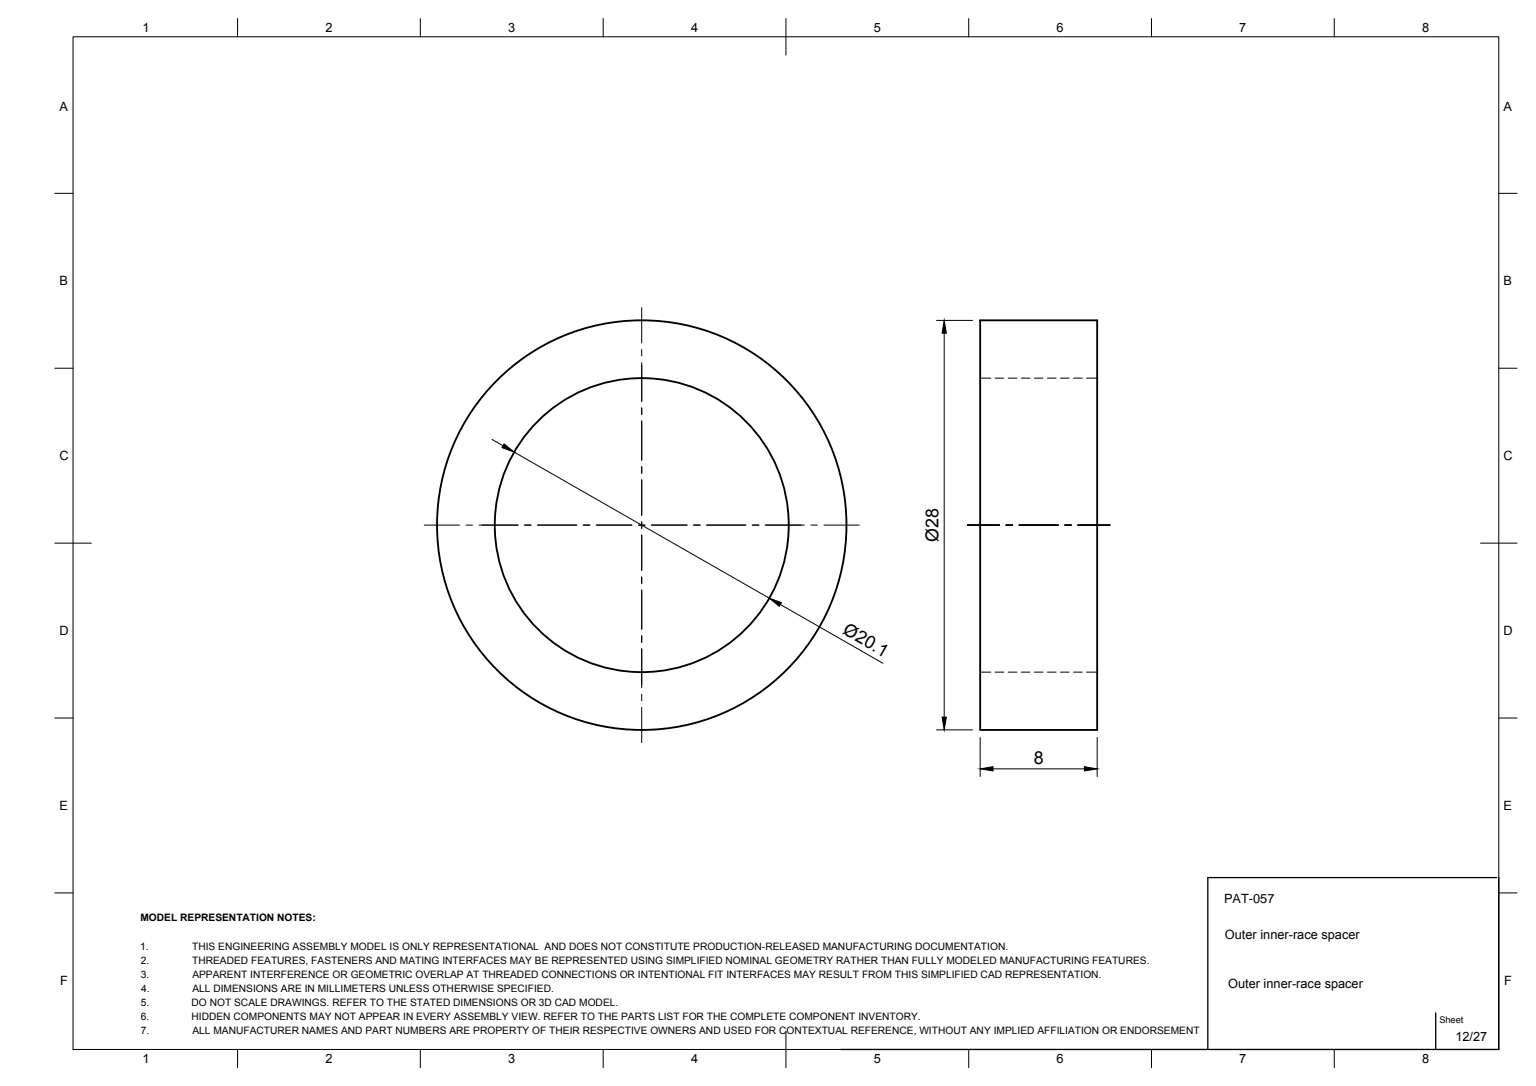
ISO-10303-21;
HEADER;
/* Generated by software containing ST-Developer
 * from STEP Tools, Inc. (www.steptools.com) 
 */

FILE_DESCRIPTION(
/* description */ ('Bearing-mounted hook block'),
/* implementation_level */ '2;1');

FILE_NAME(
/* name */ 'Outer inner-race spacer.step',
/* time_stamp */ '2026-10-28T22:30:11-07:00',
/* author */ (''),
/* organization */ (''),
/* preprocessor_version */ 'ST-DEVELOPER v20.2',
/* originating_system */ 'Autodesk Translation Framework v15.17.0.0',
/* authorisation */ '');

FILE_SCHEMA (('AUTOMOTIVE_DESIGN { 1 0 10303 214 3 1 1 }'));
ENDSEC;

DATA;
#10=MECHANICAL_DESIGN_GEOMETRIC_PRESENTATION_REPRESENTATION('',(#330),#7609);
#282=SHAPE_REPRESENTATION_RELATIONSHIP('SRR','None',#7729,#306);
#306=ADVANCED_BREP_SHAPE_REPRESENTATION('',(#362),#7589);
#330=STYLED_ITEM('',(#7917),#362);
#362=MANIFOLD_SOLID_BREP('Body1',#3926);
#451=LINE('',#6349,#681);
#452=LINE('',#6355,#682);
#681=VECTOR('',#5086,1.005);
#682=VECTOR('',#5093,1.4);
#871=CYLINDRICAL_SURFACE('',#4348,1.005);
#872=CYLINDRICAL_SURFACE('',#4351,1.4);
#951=FACE_BOUND('',#1327,.T.);
#952=FACE_BOUND('',#1329,.T.);
#1058=FACE_OUTER_BOUND('',#1324,.T.);
#1059=FACE_OUTER_BOUND('',#1325,.T.);
#1060=FACE_OUTER_BOUND('',#1326,.T.);
#1061=FACE_OUTER_BOUND('',#1328,.T.);
#1324=EDGE_LOOP('',(#2848,#2849,#2850,#2851));
#1325=EDGE_LOOP('',(#2852,#2853,#2854,#2855));
#1326=EDGE_LOOP('',(#2856));
#1327=EDGE_LOOP('',(#2857));
#1328=EDGE_LOOP('',(#2858));
#1329=EDGE_LOOP('',(#2859));
#1615=CIRCLE('',#4349,1.005);
#1616=CIRCLE('',#4350,1.005);
#1617=CIRCLE('',#4352,1.4);
#1618=CIRCLE('',#4353,1.4);
#1864=VERTEX_POINT('',#6346);
#1865=VERTEX_POINT('',#6348);
#1866=VERTEX_POINT('',#6352);
#1867=VERTEX_POINT('',#6354);
#2234=EDGE_CURVE('',#1864,#1864,#1615,.T.);
#2235=EDGE_CURVE('',#1864,#1865,#451,.T.);
#2236=EDGE_CURVE('',#1865,#1865,#1616,.T.);
#2237=EDGE_CURVE('',#1866,#1866,#1617,.T.);
#2238=EDGE_CURVE('',#1866,#1867,#452,.T.);
#2239=EDGE_CURVE('',#1867,#1867,#1618,.T.);
#2848=ORIENTED_EDGE('',*,*,#2234,.F.);
#2849=ORIENTED_EDGE('',*,*,#2235,.T.);
#2850=ORIENTED_EDGE('',*,*,#2236,.T.);
#2851=ORIENTED_EDGE('',*,*,#2235,.F.);
#2852=ORIENTED_EDGE('',*,*,#2237,.F.);
#2853=ORIENTED_EDGE('',*,*,#2238,.T.);
#2854=ORIENTED_EDGE('',*,*,#2239,.T.);
#2855=ORIENTED_EDGE('',*,*,#2238,.F.);
#2856=ORIENTED_EDGE('',*,*,#2237,.T.);
#2857=ORIENTED_EDGE('',*,*,#2234,.T.);
#2858=ORIENTED_EDGE('',*,*,#2239,.F.);
#2859=ORIENTED_EDGE('',*,*,#2236,.F.);
#3590=PLANE('',#4354);
#3591=PLANE('',#4355);
#3740=ADVANCED_FACE('',(#1058),#871,.F.);
#3741=ADVANCED_FACE('',(#1059),#872,.T.);
#3742=ADVANCED_FACE('',(#1060,#951),#3590,.T.);
#3743=ADVANCED_FACE('',(#1061,#952),#3591,.F.);
#3926=CLOSED_SHELL('',(#3740,#3741,#3742,#3743));
#4347=AXIS2_PLACEMENT_3D('',#6344,#5080,#5081);
#4348=AXIS2_PLACEMENT_3D('',#6345,#5082,#5083);
#4349=AXIS2_PLACEMENT_3D('',#6347,#5084,#5085);
#4350=AXIS2_PLACEMENT_3D('',#6350,#5087,#5088);
#4351=AXIS2_PLACEMENT_3D('',#6351,#5089,#5090);
#4352=AXIS2_PLACEMENT_3D('',#6353,#5091,#5092);
#4353=AXIS2_PLACEMENT_3D('',#6356,#5094,#5095);
#4354=AXIS2_PLACEMENT_3D('',#6357,#5096,#5097);
#4355=AXIS2_PLACEMENT_3D('',#6358,#5098,#5099);
#5080=DIRECTION('axis',(0.,0.,1.));
#5081=DIRECTION('refdir',(1.,0.,0.));
#5082=DIRECTION('center_axis',(0.,1.,0.));
#5083=DIRECTION('ref_axis',(1.,0.,0.));
#5084=DIRECTION('center_axis',(0.,-1.,0.));
#5085=DIRECTION('ref_axis',(1.,0.,0.));
#5086=DIRECTION('',(0.,-1.,0.));
#5087=DIRECTION('center_axis',(0.,-1.,0.));
#5088=DIRECTION('ref_axis',(1.,0.,0.));
#5089=DIRECTION('center_axis',(0.,1.,0.));
#5090=DIRECTION('ref_axis',(1.,0.,0.));
#5091=DIRECTION('center_axis',(0.,1.,0.));
#5092=DIRECTION('ref_axis',(1.,0.,0.));
#5093=DIRECTION('',(0.,-1.,0.));
#5094=DIRECTION('center_axis',(0.,1.,0.));
#5095=DIRECTION('ref_axis',(1.,0.,0.));
#5096=DIRECTION('center_axis',(0.,1.,0.));
#5097=DIRECTION('ref_axis',(1.,0.,0.));
#5098=DIRECTION('center_axis',(0.,1.,0.));
#5099=DIRECTION('ref_axis',(1.,0.,0.));
#6344=CARTESIAN_POINT('',(0.,0.,0.));
#6345=CARTESIAN_POINT('Origin',(0.,-2.5,12.));
#6346=CARTESIAN_POINT('',(-1.005,-1.7,12.));
#6347=CARTESIAN_POINT('Origin',(0.,-1.7,12.));
#6348=CARTESIAN_POINT('',(-1.005,-2.5,12.));
#6349=CARTESIAN_POINT('',(-1.005,-2.5,12.));
#6350=CARTESIAN_POINT('Origin',(0.,-2.5,12.));
#6351=CARTESIAN_POINT('Origin',(0.,-2.5,12.));
#6352=CARTESIAN_POINT('',(-1.4,-1.7,12.));
#6353=CARTESIAN_POINT('Origin',(0.,-1.7,12.));
#6354=CARTESIAN_POINT('',(-1.4,-2.5,12.));
#6355=CARTESIAN_POINT('',(-1.4,-2.5,12.));
#6356=CARTESIAN_POINT('Origin',(0.,-2.5,12.));
#6357=CARTESIAN_POINT('Origin',(0.,-1.7,12.));
#6358=CARTESIAN_POINT('Origin',(0.,-2.5,12.));
#7559=UNCERTAINTY_MEASURE_WITH_UNIT(LENGTH_MEASURE(0.001),#7610,
'DISTANCE_ACCURACY_VALUE',
'Maximum model space distance between geometric entities at asserted c
onnectivities');
#7579=UNCERTAINTY_MEASURE_WITH_UNIT(LENGTH_MEASURE(0.001),#7610,
'DISTANCE_ACCURACY_VALUE',
'Maximum model space distance between geometric entities at asserted c
onnectivities');
#7589=(
GEOMETRIC_REPRESENTATION_CONTEXT(3)
GLOBAL_UNCERTAINTY_ASSIGNED_CONTEXT((#7559))
GLOBAL_UNIT_ASSIGNED_CONTEXT((#7610,#7612,#7613))
REPRESENTATION_CONTEXT('','3D')
);
#7609=(
GEOMETRIC_REPRESENTATION_CONTEXT(3)
GLOBAL_UNCERTAINTY_ASSIGNED_CONTEXT((#7579))
GLOBAL_UNIT_ASSIGNED_CONTEXT((#7610,#7612,#7613))
REPRESENTATION_CONTEXT('','3D')
);
#7610=(
LENGTH_UNIT()
NAMED_UNIT(*)
SI_UNIT(.CENTI.,.METRE.)
);
#7612=(
NAMED_UNIT(*)
PLANE_ANGLE_UNIT()
SI_UNIT($,.RADIAN.)
);
#7613=(
NAMED_UNIT(*)
SI_UNIT($,.STERADIAN.)
SOLID_ANGLE_UNIT()
);
#7623=SHAPE_DEFINITION_REPRESENTATION(#7652,#7729);
#7652=PRODUCT_DEFINITION_SHAPE('',$,#7759);
#7729=SHAPE_REPRESENTATION('',(#4347),#7589);
#7749=PRODUCT_DEFINITION_CONTEXT('part definition',#7838,'design');
#7759=PRODUCT_DEFINITION('Outer inner-race spacer',
'Outer inner-race spacer',#7788,#7749);
#7788=PRODUCT_DEFINITION_FORMATION('',$,#7849);
#7838=APPLICATION_CONTEXT(
'Core Data for Automotive Mechanical Design Process');
#7839=PRODUCT_CONTEXT('part definition',#7838,'mechanical');
#7849=PRODUCT('Outer inner-race spacer','Outer inner-race spacer',
'Outer inner-race spacer',(#7839));
#7911=COLOUR_RGB('Light Blue',0.38,0.62,0.78);
#7912=FILL_AREA_STYLE_COLOUR('',#7911);
#7913=FILL_AREA_STYLE('',(#7912));
#7914=SURFACE_STYLE_FILL_AREA(#7913);
#7915=SURFACE_SIDE_STYLE('',(#7914));
#7916=SURFACE_STYLE_USAGE(.BOTH.,#7915);
#7917=PRESENTATION_STYLE_ASSIGNMENT((#7916));
ENDSEC;
END-ISO-10303-21;
